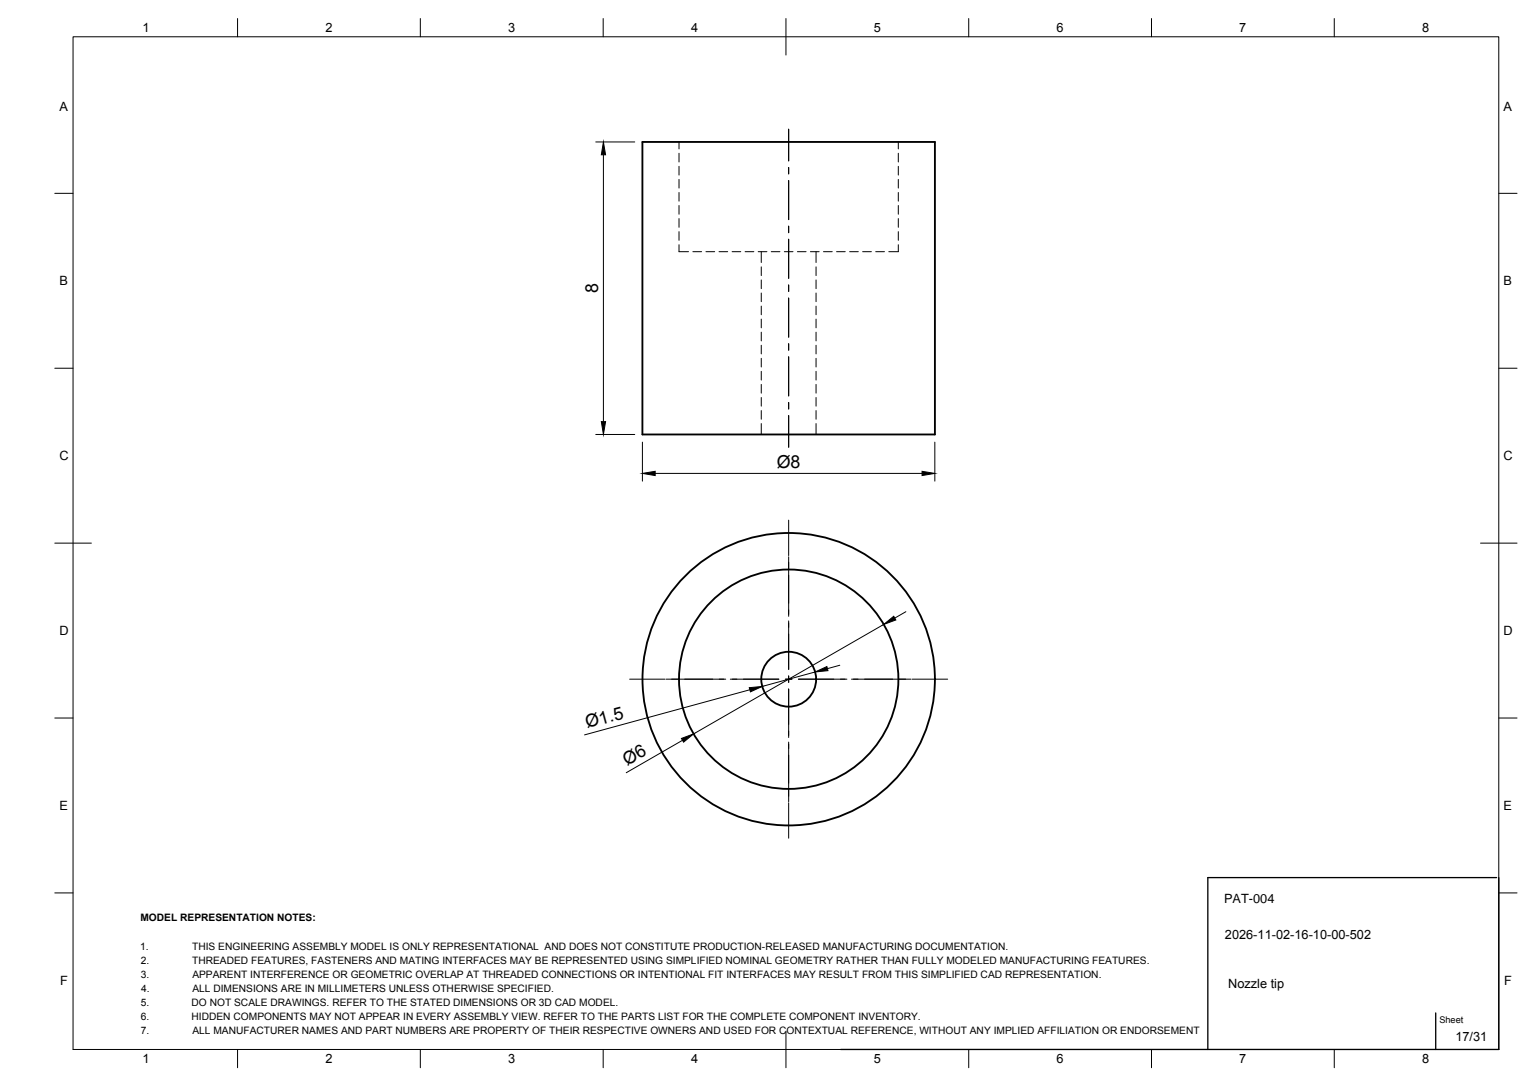
ISO-10303-21;
HEADER;
/* Generated by software containing ST-Developer
 * from STEP Tools, Inc. (www.steptools.com) 
 */

FILE_DESCRIPTION(
/* description */ ('Air blow-off nozzle station'),
/* implementation_level */ '2;1');

FILE_NAME(
/* name */ 'Nozzle tip.step',
/* time_stamp */ '2026-10-27T10:53:54-07:00',
/* author */ (''),
/* organization */ (''),
/* preprocessor_version */ 'ST-DEVELOPER v20.2',
/* originating_system */ 'Autodesk Translation Framework v15.17.0.0',
/* authorisation */ '');

FILE_SCHEMA (('AUTOMOTIVE_DESIGN { 1 0 10303 214 3 1 1 }'));
ENDSEC;

DATA;
#10=MECHANICAL_DESIGN_GEOMETRIC_PRESENTATION_REPRESENTATION('',(#253),#7897);
#203=SHAPE_REPRESENTATION_RELATIONSHIP('SRR','None',#8018,#228);
#228=ADVANCED_BREP_SHAPE_REPRESENTATION('',(#276),#7885);
#253=STYLED_ITEM('',(#8213),#276);
#276=MANIFOLD_SOLID_BREP('Body1',#4304);
#341=FACE_BOUND('',#1049,.T.);
#342=FACE_BOUND('',#1053,.T.);
#343=FACE_BOUND('',#1055,.T.);
#508=PLANE('',#4929);
#509=PLANE('',#4936);
#510=PLANE('',#4937);
#735=FACE_OUTER_BOUND('',#1047,.T.);
#736=FACE_OUTER_BOUND('',#1048,.T.);
#737=FACE_OUTER_BOUND('',#1050,.T.);
#738=FACE_OUTER_BOUND('',#1051,.T.);
#739=FACE_OUTER_BOUND('',#1052,.T.);
#740=FACE_OUTER_BOUND('',#1054,.T.);
#1047=EDGE_LOOP('',(#3757,#3758,#3759,#3760));
#1048=EDGE_LOOP('',(#3761));
#1049=EDGE_LOOP('',(#3762));
#1050=EDGE_LOOP('',(#3763,#3764,#3765,#3766));
#1051=EDGE_LOOP('',(#3767,#3768,#3769,#3770));
#1052=EDGE_LOOP('',(#3771));
#1053=EDGE_LOOP('',(#3772));
#1054=EDGE_LOOP('',(#3773));
#1055=EDGE_LOOP('',(#3774));
#1447=LINE('',#7577,#1801);
#1448=LINE('',#7584,#1802);
#1449=LINE('',#7590,#1803);
#1801=VECTOR('',#6059,0.3);
#1802=VECTOR('',#6068,0.0750000000000002);
#1803=VECTOR('',#6075,0.4);
#1951=CIRCLE('',#4927,0.3);
#1952=CIRCLE('',#4928,0.3);
#1953=CIRCLE('',#4930,0.0750000000000002);
#1954=CIRCLE('',#4932,0.0750000000000002);
#1955=CIRCLE('',#4934,0.4);
#1956=CIRCLE('',#4935,0.4);
#2296=VERTEX_POINT('',#7574);
#2297=VERTEX_POINT('',#7576);
#2298=VERTEX_POINT('',#7580);
#2299=VERTEX_POINT('',#7583);
#2300=VERTEX_POINT('',#7587);
#2301=VERTEX_POINT('',#7589);
#2796=EDGE_CURVE('',#2296,#2296,#1951,.T.);
#2797=EDGE_CURVE('',#2296,#2297,#1447,.T.);
#2798=EDGE_CURVE('',#2297,#2297,#1952,.T.);
#2799=EDGE_CURVE('',#2298,#2298,#1953,.T.);
#2800=EDGE_CURVE('',#2298,#2299,#1448,.T.);
#2801=EDGE_CURVE('',#2299,#2299,#1954,.T.);
#2802=EDGE_CURVE('',#2300,#2300,#1955,.T.);
#2803=EDGE_CURVE('',#2300,#2301,#1449,.T.);
#2804=EDGE_CURVE('',#2301,#2301,#1956,.T.);
#3757=ORIENTED_EDGE('',*,*,#2796,.F.);
#3758=ORIENTED_EDGE('',*,*,#2797,.T.);
#3759=ORIENTED_EDGE('',*,*,#2798,.F.);
#3760=ORIENTED_EDGE('',*,*,#2797,.F.);
#3761=ORIENTED_EDGE('',*,*,#2796,.T.);
#3762=ORIENTED_EDGE('',*,*,#2799,.F.);
#3763=ORIENTED_EDGE('',*,*,#2799,.T.);
#3764=ORIENTED_EDGE('',*,*,#2800,.T.);
#3765=ORIENTED_EDGE('',*,*,#2801,.T.);
#3766=ORIENTED_EDGE('',*,*,#2800,.F.);
#3767=ORIENTED_EDGE('',*,*,#2802,.F.);
#3768=ORIENTED_EDGE('',*,*,#2803,.T.);
#3769=ORIENTED_EDGE('',*,*,#2804,.T.);
#3770=ORIENTED_EDGE('',*,*,#2803,.F.);
#3771=ORIENTED_EDGE('',*,*,#2802,.T.);
#3772=ORIENTED_EDGE('',*,*,#2798,.T.);
#3773=ORIENTED_EDGE('',*,*,#2804,.F.);
#3774=ORIENTED_EDGE('',*,*,#2801,.F.);
#4003=CYLINDRICAL_SURFACE('',#4926,0.3);
#4004=CYLINDRICAL_SURFACE('',#4931,0.0750000000000002);
#4005=CYLINDRICAL_SURFACE('',#4933,0.4);
#4225=ADVANCED_FACE('',(#735),#4003,.F.);
#4226=ADVANCED_FACE('',(#736,#341),#508,.T.);
#4227=ADVANCED_FACE('',(#737),#4004,.F.);
#4228=ADVANCED_FACE('',(#738),#4005,.T.);
#4229=ADVANCED_FACE('',(#739,#342),#509,.T.);
#4230=ADVANCED_FACE('',(#740,#343),#510,.F.);
#4304=CLOSED_SHELL('',(#4225,#4226,#4227,#4228,#4229,#4230));
#4925=AXIS2_PLACEMENT_3D('',#7572,#6053,#6054);
#4926=AXIS2_PLACEMENT_3D('',#7573,#6055,#6056);
#4927=AXIS2_PLACEMENT_3D('',#7575,#6057,#6058);
#4928=AXIS2_PLACEMENT_3D('',#7578,#6060,#6061);
#4929=AXIS2_PLACEMENT_3D('',#7579,#6062,#6063);
#4930=AXIS2_PLACEMENT_3D('',#7581,#6064,#6065);
#4931=AXIS2_PLACEMENT_3D('',#7582,#6066,#6067);
#4932=AXIS2_PLACEMENT_3D('',#7585,#6069,#6070);
#4933=AXIS2_PLACEMENT_3D('',#7586,#6071,#6072);
#4934=AXIS2_PLACEMENT_3D('',#7588,#6073,#6074);
#4935=AXIS2_PLACEMENT_3D('',#7591,#6076,#6077);
#4936=AXIS2_PLACEMENT_3D('',#7592,#6078,#6079);
#4937=AXIS2_PLACEMENT_3D('',#7593,#6080,#6081);
#6053=DIRECTION('axis',(0.,0.,1.));
#6054=DIRECTION('refdir',(1.,0.,0.));
#6055=DIRECTION('center_axis',(0.,1.,0.));
#6056=DIRECTION('ref_axis',(1.,0.,0.));
#6057=DIRECTION('center_axis',(0.,1.,0.));
#6058=DIRECTION('ref_axis',(1.,0.,0.));
#6059=DIRECTION('',(0.,1.,0.));
#6060=DIRECTION('center_axis',(0.,-1.,0.));
#6061=DIRECTION('ref_axis',(1.,0.,0.));
#6062=DIRECTION('center_axis',(0.,1.,0.));
#6063=DIRECTION('ref_axis',(1.,0.,0.));
#6064=DIRECTION('center_axis',(0.,1.,0.));
#6065=DIRECTION('ref_axis',(1.,0.,0.));
#6066=DIRECTION('center_axis',(0.,1.,0.));
#6067=DIRECTION('ref_axis',(1.,0.,0.));
#6068=DIRECTION('',(0.,-1.,0.));
#6069=DIRECTION('center_axis',(0.,-1.,0.));
#6070=DIRECTION('ref_axis',(1.,0.,0.));
#6071=DIRECTION('center_axis',(0.,1.,0.));
#6072=DIRECTION('ref_axis',(1.,0.,0.));
#6073=DIRECTION('center_axis',(0.,1.,0.));
#6074=DIRECTION('ref_axis',(1.,0.,0.));
#6075=DIRECTION('',(0.,-1.,0.));
#6076=DIRECTION('center_axis',(0.,1.,0.));
#6077=DIRECTION('ref_axis',(1.,0.,0.));
#6078=DIRECTION('center_axis',(0.,1.,0.));
#6079=DIRECTION('ref_axis',(1.,0.,0.));
#6080=DIRECTION('center_axis',(0.,1.,0.));
#6081=DIRECTION('ref_axis',(1.,0.,0.));
#7572=CARTESIAN_POINT('',(0.,0.,0.));
#7573=CARTESIAN_POINT('Origin',(-3.,-7.2,23.));
#7574=CARTESIAN_POINT('',(-3.3,-7.2,23.));
#7575=CARTESIAN_POINT('Origin',(-3.,-7.2,23.));
#7576=CARTESIAN_POINT('',(-3.3,-6.9,23.));
#7577=CARTESIAN_POINT('',(-3.3,-7.2,23.));
#7578=CARTESIAN_POINT('Origin',(-3.,-6.9,23.));
#7579=CARTESIAN_POINT('Origin',(-3.,-7.2,23.));
#7580=CARTESIAN_POINT('',(-3.075,-7.2,23.));
#7581=CARTESIAN_POINT('Origin',(-3.,-7.2,23.));
#7582=CARTESIAN_POINT('Origin',(-3.,-7.7,23.));
#7583=CARTESIAN_POINT('',(-3.075,-7.7,23.));
#7584=CARTESIAN_POINT('',(-3.075,-7.7,23.));
#7585=CARTESIAN_POINT('Origin',(-3.,-7.7,23.));
#7586=CARTESIAN_POINT('Origin',(-3.,-7.7,23.));
#7587=CARTESIAN_POINT('',(-3.4,-6.9,23.));
#7588=CARTESIAN_POINT('Origin',(-3.,-6.9,23.));
#7589=CARTESIAN_POINT('',(-3.4,-7.7,23.));
#7590=CARTESIAN_POINT('',(-3.4,-7.7,23.));
#7591=CARTESIAN_POINT('Origin',(-3.,-7.7,23.));
#7592=CARTESIAN_POINT('Origin',(-3.,-6.9,23.));
#7593=CARTESIAN_POINT('Origin',(-3.,-7.7,23.));
#7853=UNCERTAINTY_MEASURE_WITH_UNIT(LENGTH_MEASURE(0.001),#7898,
'DISTANCE_ACCURACY_VALUE',
'Maximum model space distance between geometric entities at asserted c
onnectivities');
#7865=UNCERTAINTY_MEASURE_WITH_UNIT(LENGTH_MEASURE(0.001),#7898,
'DISTANCE_ACCURACY_VALUE',
'Maximum model space distance between geometric entities at asserted c
onnectivities');
#7885=(
GEOMETRIC_REPRESENTATION_CONTEXT(3)
GLOBAL_UNCERTAINTY_ASSIGNED_CONTEXT((#7853))
GLOBAL_UNIT_ASSIGNED_CONTEXT((#7898,#7900,#7901))
REPRESENTATION_CONTEXT('','3D')
);
#7897=(
GEOMETRIC_REPRESENTATION_CONTEXT(3)
GLOBAL_UNCERTAINTY_ASSIGNED_CONTEXT((#7865))
GLOBAL_UNIT_ASSIGNED_CONTEXT((#7898,#7900,#7901))
REPRESENTATION_CONTEXT('','3D')
);
#7898=(
LENGTH_UNIT()
NAMED_UNIT(*)
SI_UNIT(.CENTI.,.METRE.)
);
#7900=(
NAMED_UNIT(*)
PLANE_ANGLE_UNIT()
SI_UNIT($,.RADIAN.)
);
#7901=(
NAMED_UNIT(*)
SI_UNIT($,.STERADIAN.)
SOLID_ANGLE_UNIT()
);
#7921=SHAPE_DEFINITION_REPRESENTATION(#7969,#8018);
#7969=PRODUCT_DEFINITION_SHAPE('',$,#8050);
#8018=SHAPE_REPRESENTATION('',(#4925),#7885);
#8030=PRODUCT_DEFINITION_CONTEXT('part definition',#8125,'design');
#8050=PRODUCT_DEFINITION('Nozzle tip','Nozzle tip',#8081,#8030);
#8081=PRODUCT_DEFINITION_FORMATION('',$,#8146);
#8125=APPLICATION_CONTEXT(
'Core Data for Automotive Mechanical Design Process');
#8126=PRODUCT_CONTEXT('part definition',#8125,'mechanical');
#8146=PRODUCT('Nozzle tip','Nozzle tip','Nozzle tip',(#8126));
#8207=COLOUR_RGB('Sky Blue',0.24,0.69,0.87);
#8208=FILL_AREA_STYLE_COLOUR('',#8207);
#8209=FILL_AREA_STYLE('',(#8208));
#8210=SURFACE_STYLE_FILL_AREA(#8209);
#8211=SURFACE_SIDE_STYLE('',(#8210));
#8212=SURFACE_STYLE_USAGE(.BOTH.,#8211);
#8213=PRESENTATION_STYLE_ASSIGNMENT((#8212));
ENDSEC;
END-ISO-10303-21;
